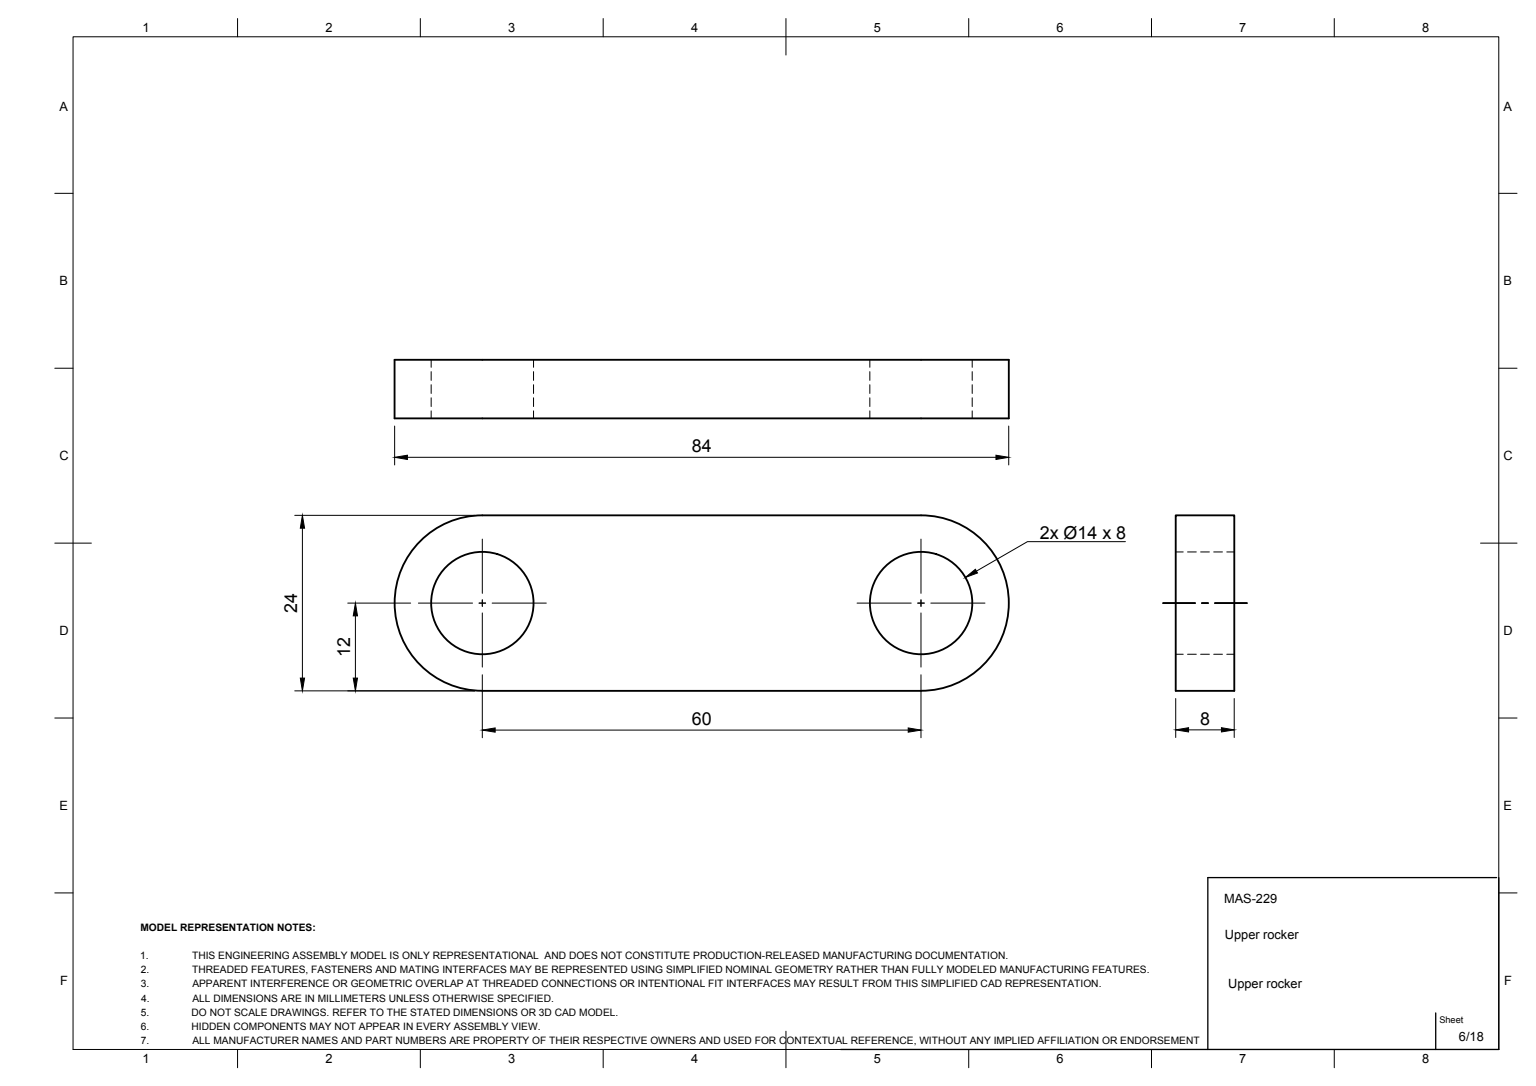
ISO-10303-21;
HEADER;
/* Generated by software containing ST-Developer
 * from STEP Tools, Inc. (www.steptools.com) 
 */

FILE_DESCRIPTION(
/* description */ ('Independently dimensioned six-bar single-leg walking-linkage demonstr
ator. Whole-mm20 crank,60 upper rocker,80/120 ternary coupler,120 lowe
r rocker,140 knee pitch and260 toe reach; ground pivots0/0,60/0,40/60.
 Seven native revolutes close both loops. Four reused native library f
amilies, fully retained shared pins and layered real spacer stacks, bo
nded rubber toe. Benchtop reference mechanism; no complete vehicle, lo
ad, gait stability, adhesive, weld, fit or life rating.'),
/* implementation_level */ '2;1');

FILE_NAME(
/* name */ 'Upper rocker.step',
/* time_stamp */ '2026-11-09T20:33:14-08:00',
/* author */ (''),
/* organization */ (''),
/* preprocessor_version */ 'ST-DEVELOPER v20.2',
/* originating_system */ 'Autodesk Translation Framework v15.17.0.0',
/* authorisation */ '');

FILE_SCHEMA (('AUTOMOTIVE_DESIGN { 1 0 10303 214 3 1 1 }'));
ENDSEC;

DATA;
#10=MECHANICAL_DESIGN_GEOMETRIC_PRESENTATION_REPRESENTATION('',(#258),#4048);
#222=SHAPE_REPRESENTATION_RELATIONSHIP('SRR','None',#4146,#240);
#240=ADVANCED_BREP_SHAPE_REPRESENTATION('',(#276),#4033);
#258=STYLED_ITEM('',(#4245),#276);
#276=MANIFOLD_SOLID_BREP('Body1',#2147);
#309=FACE_BOUND('',#595,.T.);
#310=FACE_BOUND('',#596,.T.);
#311=FACE_BOUND('',#598,.T.);
#312=FACE_BOUND('',#599,.T.);
#366=PLANE('',#2423);
#367=PLANE('',#2427);
#368=PLANE('',#2431);
#369=PLANE('',#2432);
#444=FACE_OUTER_BOUND('',#588,.T.);
#445=FACE_OUTER_BOUND('',#589,.T.);
#446=FACE_OUTER_BOUND('',#590,.T.);
#447=FACE_OUTER_BOUND('',#591,.T.);
#448=FACE_OUTER_BOUND('',#592,.T.);
#449=FACE_OUTER_BOUND('',#593,.T.);
#450=FACE_OUTER_BOUND('',#594,.T.);
#451=FACE_OUTER_BOUND('',#597,.T.);
#588=EDGE_LOOP('',(#1623,#1624,#1625,#1626));
#589=EDGE_LOOP('',(#1627,#1628,#1629,#1630));
#590=EDGE_LOOP('',(#1631,#1632,#1633,#1634));
#591=EDGE_LOOP('',(#1635,#1636,#1637,#1638));
#592=EDGE_LOOP('',(#1639,#1640,#1641,#1642));
#593=EDGE_LOOP('',(#1643,#1644,#1645,#1646));
#594=EDGE_LOOP('',(#1647,#1648,#1649,#1650));
#595=EDGE_LOOP('',(#1651));
#596=EDGE_LOOP('',(#1652));
#597=EDGE_LOOP('',(#1653,#1654,#1655,#1656));
#598=EDGE_LOOP('',(#1657));
#599=EDGE_LOOP('',(#1658));
#771=LINE('',#3569,#896);
#772=LINE('',#3575,#897);
#773=LINE('',#3580,#898);
#774=LINE('',#3582,#899);
#775=LINE('',#3584,#900);
#776=LINE('',#3585,#901);
#777=LINE('',#3591,#902);
#778=LINE('',#3594,#903);
#779=LINE('',#3596,#904);
#780=LINE('',#3597,#905);
#896=VECTOR('',#2834,7.);
#897=VECTOR('',#2841,7.);
#898=VECTOR('',#2846,10.);
#899=VECTOR('',#2847,10.);
#900=VECTOR('',#2848,10.);
#901=VECTOR('',#2849,10.);
#902=VECTOR('',#2856,10.);
#903=VECTOR('',#2859,10.);
#904=VECTOR('',#2860,10.);
#905=VECTOR('',#2861,10.);
#996=CIRCLE('',#2418,7.);
#997=CIRCLE('',#2419,7.);
#998=CIRCLE('',#2421,7.);
#999=CIRCLE('',#2422,7.);
#1000=CIRCLE('',#2425,12.);
#1001=CIRCLE('',#2426,12.);
#1002=CIRCLE('',#2429,12.);
#1003=CIRCLE('',#2430,12.);
#1134=VERTEX_POINT('',#3566);
#1135=VERTEX_POINT('',#3568);
#1136=VERTEX_POINT('',#3572);
#1137=VERTEX_POINT('',#3574);
#1138=VERTEX_POINT('',#3578);
#1139=VERTEX_POINT('',#3579);
#1140=VERTEX_POINT('',#3581);
#1141=VERTEX_POINT('',#3583);
#1142=VERTEX_POINT('',#3587);
#1143=VERTEX_POINT('',#3589);
#1144=VERTEX_POINT('',#3593);
#1145=VERTEX_POINT('',#3595);
#1315=EDGE_CURVE('',#1134,#1134,#996,.T.);
#1316=EDGE_CURVE('',#1134,#1135,#771,.T.);
#1317=EDGE_CURVE('',#1135,#1135,#997,.T.);
#1318=EDGE_CURVE('',#1136,#1136,#998,.T.);
#1319=EDGE_CURVE('',#1136,#1137,#772,.T.);
#1320=EDGE_CURVE('',#1137,#1137,#999,.T.);
#1321=EDGE_CURVE('',#1138,#1139,#773,.T.);
#1322=EDGE_CURVE('',#1139,#1140,#774,.T.);
#1323=EDGE_CURVE('',#1141,#1140,#775,.T.);
#1324=EDGE_CURVE('',#1138,#1141,#776,.T.);
#1325=EDGE_CURVE('',#1142,#1138,#1000,.T.);
#1326=EDGE_CURVE('',#1143,#1141,#1001,.T.);
#1327=EDGE_CURVE('',#1142,#1143,#777,.T.);
#1328=EDGE_CURVE('',#1144,#1142,#778,.T.);
#1329=EDGE_CURVE('',#1145,#1143,#779,.T.);
#1330=EDGE_CURVE('',#1144,#1145,#780,.T.);
#1331=EDGE_CURVE('',#1139,#1144,#1002,.T.);
#1332=EDGE_CURVE('',#1140,#1145,#1003,.T.);
#1623=ORIENTED_EDGE('',*,*,#1315,.F.);
#1624=ORIENTED_EDGE('',*,*,#1316,.T.);
#1625=ORIENTED_EDGE('',*,*,#1317,.F.);
#1626=ORIENTED_EDGE('',*,*,#1316,.F.);
#1627=ORIENTED_EDGE('',*,*,#1318,.F.);
#1628=ORIENTED_EDGE('',*,*,#1319,.T.);
#1629=ORIENTED_EDGE('',*,*,#1320,.F.);
#1630=ORIENTED_EDGE('',*,*,#1319,.F.);
#1631=ORIENTED_EDGE('',*,*,#1321,.T.);
#1632=ORIENTED_EDGE('',*,*,#1322,.T.);
#1633=ORIENTED_EDGE('',*,*,#1323,.F.);
#1634=ORIENTED_EDGE('',*,*,#1324,.F.);
#1635=ORIENTED_EDGE('',*,*,#1325,.T.);
#1636=ORIENTED_EDGE('',*,*,#1324,.T.);
#1637=ORIENTED_EDGE('',*,*,#1326,.F.);
#1638=ORIENTED_EDGE('',*,*,#1327,.F.);
#1639=ORIENTED_EDGE('',*,*,#1328,.T.);
#1640=ORIENTED_EDGE('',*,*,#1327,.T.);
#1641=ORIENTED_EDGE('',*,*,#1329,.F.);
#1642=ORIENTED_EDGE('',*,*,#1330,.F.);
#1643=ORIENTED_EDGE('',*,*,#1331,.T.);
#1644=ORIENTED_EDGE('',*,*,#1330,.T.);
#1645=ORIENTED_EDGE('',*,*,#1332,.F.);
#1646=ORIENTED_EDGE('',*,*,#1322,.F.);
#1647=ORIENTED_EDGE('',*,*,#1332,.T.);
#1648=ORIENTED_EDGE('',*,*,#1329,.T.);
#1649=ORIENTED_EDGE('',*,*,#1326,.T.);
#1650=ORIENTED_EDGE('',*,*,#1323,.T.);
#1651=ORIENTED_EDGE('',*,*,#1315,.T.);
#1652=ORIENTED_EDGE('',*,*,#1318,.T.);
#1653=ORIENTED_EDGE('',*,*,#1331,.F.);
#1654=ORIENTED_EDGE('',*,*,#1321,.F.);
#1655=ORIENTED_EDGE('',*,*,#1325,.F.);
#1656=ORIENTED_EDGE('',*,*,#1328,.F.);
#1657=ORIENTED_EDGE('',*,*,#1317,.T.);
#1658=ORIENTED_EDGE('',*,*,#1320,.T.);
#1974=CYLINDRICAL_SURFACE('',#2417,7.);
#1975=CYLINDRICAL_SURFACE('',#2420,7.);
#1976=CYLINDRICAL_SURFACE('',#2424,12.);
#1977=CYLINDRICAL_SURFACE('',#2428,12.);
#2047=ADVANCED_FACE('',(#444),#1974,.F.);
#2048=ADVANCED_FACE('',(#445),#1975,.F.);
#2049=ADVANCED_FACE('',(#446),#366,.T.);
#2050=ADVANCED_FACE('',(#447),#1976,.T.);
#2051=ADVANCED_FACE('',(#448),#367,.T.);
#2052=ADVANCED_FACE('',(#449),#1977,.T.);
#2053=ADVANCED_FACE('',(#450,#309,#310),#368,.T.);
#2054=ADVANCED_FACE('',(#451,#311,#312),#369,.F.);
#2147=CLOSED_SHELL('',(#2047,#2048,#2049,#2050,#2051,#2052,#2053,#2054));
#2416=AXIS2_PLACEMENT_3D('',#3564,#2828,#2829);
#2417=AXIS2_PLACEMENT_3D('',#3565,#2830,#2831);
#2418=AXIS2_PLACEMENT_3D('',#3567,#2832,#2833);
#2419=AXIS2_PLACEMENT_3D('',#3570,#2835,#2836);
#2420=AXIS2_PLACEMENT_3D('',#3571,#2837,#2838);
#2421=AXIS2_PLACEMENT_3D('',#3573,#2839,#2840);
#2422=AXIS2_PLACEMENT_3D('',#3576,#2842,#2843);
#2423=AXIS2_PLACEMENT_3D('',#3577,#2844,#2845);
#2424=AXIS2_PLACEMENT_3D('',#3586,#2850,#2851);
#2425=AXIS2_PLACEMENT_3D('',#3588,#2852,#2853);
#2426=AXIS2_PLACEMENT_3D('',#3590,#2854,#2855);
#2427=AXIS2_PLACEMENT_3D('',#3592,#2857,#2858);
#2428=AXIS2_PLACEMENT_3D('',#3598,#2862,#2863);
#2429=AXIS2_PLACEMENT_3D('',#3599,#2864,#2865);
#2430=AXIS2_PLACEMENT_3D('',#3600,#2866,#2867);
#2431=AXIS2_PLACEMENT_3D('',#3601,#2868,#2869);
#2432=AXIS2_PLACEMENT_3D('',#3602,#2870,#2871);
#2828=DIRECTION('axis',(0.,0.,1.));
#2829=DIRECTION('refdir',(1.,0.,0.));
#2830=DIRECTION('center_axis',(0.,0.,-1.));
#2831=DIRECTION('ref_axis',(1.,0.,0.));
#2832=DIRECTION('center_axis',(0.,0.,-1.));
#2833=DIRECTION('ref_axis',(1.,0.,0.));
#2834=DIRECTION('',(0.,0.,-1.));
#2835=DIRECTION('center_axis',(0.,0.,1.));
#2836=DIRECTION('ref_axis',(1.,0.,0.));
#2837=DIRECTION('center_axis',(0.,0.,-1.));
#2838=DIRECTION('ref_axis',(1.,0.,0.));
#2839=DIRECTION('center_axis',(0.,0.,-1.));
#2840=DIRECTION('ref_axis',(1.,0.,0.));
#2841=DIRECTION('',(0.,0.,-1.));
#2842=DIRECTION('center_axis',(0.,0.,1.));
#2843=DIRECTION('ref_axis',(1.,0.,0.));
#2844=DIRECTION('center_axis',(0.,1.,0.));
#2845=DIRECTION('ref_axis',(-1.,0.,0.));
#2846=DIRECTION('',(-1.,0.,0.));
#2847=DIRECTION('',(0.,0.,1.));
#2848=DIRECTION('',(-1.,0.,0.));
#2849=DIRECTION('',(0.,0.,1.));
#2850=DIRECTION('center_axis',(0.,0.,1.));
#2851=DIRECTION('ref_axis',(0.,-1.,0.));
#2852=DIRECTION('center_axis',(0.,0.,1.));
#2853=DIRECTION('ref_axis',(0.,-1.,0.));
#2854=DIRECTION('center_axis',(0.,0.,1.));
#2855=DIRECTION('ref_axis',(0.,-1.,0.));
#2856=DIRECTION('',(0.,0.,1.));
#2857=DIRECTION('center_axis',(0.,-1.,0.));
#2858=DIRECTION('ref_axis',(1.,0.,0.));
#2859=DIRECTION('',(1.,0.,0.));
#2860=DIRECTION('',(1.,0.,0.));
#2861=DIRECTION('',(0.,0.,1.));
#2862=DIRECTION('center_axis',(0.,0.,1.));
#2863=DIRECTION('ref_axis',(0.,1.,0.));
#2864=DIRECTION('center_axis',(0.,0.,1.));
#2865=DIRECTION('ref_axis',(0.,1.,0.));
#2866=DIRECTION('center_axis',(0.,0.,1.));
#2867=DIRECTION('ref_axis',(0.,1.,0.));
#2868=DIRECTION('center_axis',(0.,0.,1.));
#2869=DIRECTION('ref_axis',(1.,0.,0.));
#2870=DIRECTION('center_axis',(0.,0.,1.));
#2871=DIRECTION('ref_axis',(1.,0.,0.));
#3564=CARTESIAN_POINT('',(0.,0.,0.));
#3565=CARTESIAN_POINT('Origin',(0.,0.,4.));
#3566=CARTESIAN_POINT('',(-7.,8.57252759403147E-16,8.));
#3567=CARTESIAN_POINT('Origin',(0.,0.,8.));
#3568=CARTESIAN_POINT('',(-7.,8.57252759403147E-16,0.));
#3569=CARTESIAN_POINT('',(-7.,8.57252759403147E-16,4.));
#3570=CARTESIAN_POINT('Origin',(0.,0.,0.));
#3571=CARTESIAN_POINT('Origin',(60.,0.,4.));
#3572=CARTESIAN_POINT('',(53.,8.57252759403147E-16,8.));
#3573=CARTESIAN_POINT('Origin',(60.,0.,8.));
#3574=CARTESIAN_POINT('',(53.,8.57252759403147E-16,0.));
#3575=CARTESIAN_POINT('',(53.,8.57252759403147E-16,4.));
#3576=CARTESIAN_POINT('Origin',(60.,0.,0.));
#3577=CARTESIAN_POINT('Origin',(60.,12.,0.));
#3578=CARTESIAN_POINT('',(60.,12.,0.));
#3579=CARTESIAN_POINT('',(0.,12.,0.));
#3580=CARTESIAN_POINT('',(60.,12.,0.));
#3581=CARTESIAN_POINT('',(0.,12.,8.));
#3582=CARTESIAN_POINT('',(0.,12.,0.));
#3583=CARTESIAN_POINT('',(60.,12.,8.));
#3584=CARTESIAN_POINT('',(60.,12.,8.));
#3585=CARTESIAN_POINT('',(60.,12.,0.));
#3586=CARTESIAN_POINT('Origin',(60.,0.,0.));
#3587=CARTESIAN_POINT('',(60.,-12.,0.));
#3588=CARTESIAN_POINT('Origin',(60.,0.,0.));
#3589=CARTESIAN_POINT('',(60.,-12.,8.));
#3590=CARTESIAN_POINT('Origin',(60.,0.,8.));
#3591=CARTESIAN_POINT('',(60.,-12.,0.));
#3592=CARTESIAN_POINT('Origin',(0.,-12.,0.));
#3593=CARTESIAN_POINT('',(-1.46957615897682E-15,-12.,0.));
#3594=CARTESIAN_POINT('',(0.,-12.,0.));
#3595=CARTESIAN_POINT('',(-1.46957615897682E-15,-12.,8.));
#3596=CARTESIAN_POINT('',(0.,-12.,8.));
#3597=CARTESIAN_POINT('',(-1.46957615897682E-15,-12.,0.));
#3598=CARTESIAN_POINT('Origin',(0.,0.,0.));
#3599=CARTESIAN_POINT('Origin',(0.,0.,0.));
#3600=CARTESIAN_POINT('Origin',(0.,0.,8.));
#3601=CARTESIAN_POINT('Origin',(30.,0.,8.));
#3602=CARTESIAN_POINT('Origin',(30.,0.,0.));
#4013=UNCERTAINTY_MEASURE_WITH_UNIT(LENGTH_MEASURE(0.01),#4049,
'DISTANCE_ACCURACY_VALUE',
'Maximum model space distance between geometric entities at asserted c
onnectivities');
#4028=UNCERTAINTY_MEASURE_WITH_UNIT(LENGTH_MEASURE(0.01),#4049,
'DISTANCE_ACCURACY_VALUE',
'Maximum model space distance between geometric entities at asserted c
onnectivities');
#4033=(
GEOMETRIC_REPRESENTATION_CONTEXT(3)
GLOBAL_UNCERTAINTY_ASSIGNED_CONTEXT((#4013))
GLOBAL_UNIT_ASSIGNED_CONTEXT((#4049,#4051,#4052))
REPRESENTATION_CONTEXT('','3D')
);
#4048=(
GEOMETRIC_REPRESENTATION_CONTEXT(3)
GLOBAL_UNCERTAINTY_ASSIGNED_CONTEXT((#4028))
GLOBAL_UNIT_ASSIGNED_CONTEXT((#4049,#4051,#4052))
REPRESENTATION_CONTEXT('','3D')
);
#4049=(
LENGTH_UNIT()
NAMED_UNIT(*)
SI_UNIT(.MILLI.,.METRE.)
);
#4051=(
NAMED_UNIT(*)
PLANE_ANGLE_UNIT()
SI_UNIT($,.RADIAN.)
);
#4052=(
NAMED_UNIT(*)
SI_UNIT($,.STERADIAN.)
SOLID_ANGLE_UNIT()
);
#4057=SHAPE_DEFINITION_REPRESENTATION(#4076,#4146);
#4076=PRODUCT_DEFINITION_SHAPE('',$,#4166);
#4146=SHAPE_REPRESENTATION('',(#2416),#4033);
#4161=PRODUCT_DEFINITION_CONTEXT('part definition',#4220,'design');
#4166=PRODUCT_DEFINITION('Upper rocker','Upper rocker',#4185,#4161);
#4185=PRODUCT_DEFINITION_FORMATION('',$,#4226);
#4220=APPLICATION_CONTEXT(
'Core Data for Automotive Mechanical Design Process');
#4221=PRODUCT_CONTEXT('part definition',#4220,'mechanical');
#4226=PRODUCT('Upper rocker','Upper rocker',$,(#4221));
#4245=PRESENTATION_STYLE_ASSIGNMENT((#4259));
#4259=SURFACE_STYLE_USAGE(.BOTH.,#4273);
#4273=SURFACE_SIDE_STYLE('',(#4287));
#4287=SURFACE_STYLE_FILL_AREA(#4301);
#4301=FILL_AREA_STYLE('Upper rocker finish',(#4315));
#4315=FILL_AREA_STYLE_COLOUR('Upper rocker finish',#4329);
#4329=COLOUR_RGB('Upper rocker finish',0.317647058823529,0.686274509803922,
0.890196078431372);
ENDSEC;
END-ISO-10303-21;
